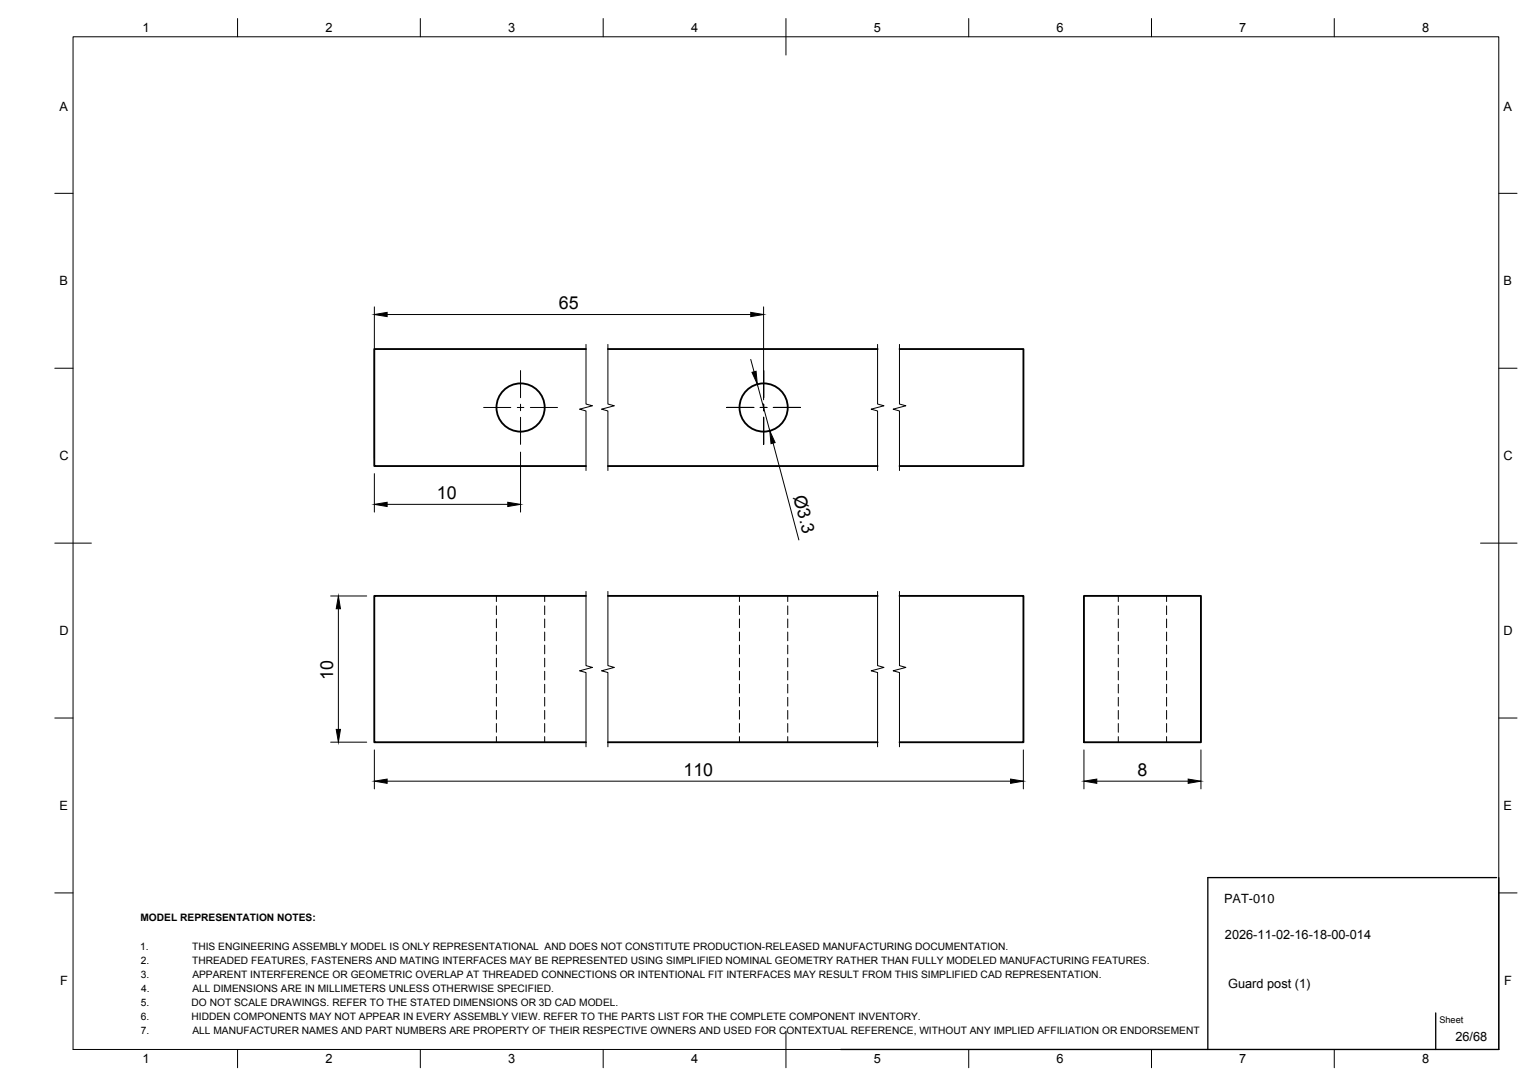
ISO-10303-21;
HEADER;
/* Generated by software containing ST-Developer
 * from STEP Tools, Inc. (www.steptools.com) 
 */

FILE_DESCRIPTION(
/* description */ ('Belt conveyor head drive unit'),
/* implementation_level */ '2;1');

FILE_NAME(
/* name */ 'Guard post (1).step',
/* time_stamp */ '2026-10-28T03:26:19-07:00',
/* author */ (''),
/* organization */ (''),
/* preprocessor_version */ 'ST-DEVELOPER v20.2',
/* originating_system */ 'Autodesk Translation Framework v15.17.0.0',
/* authorisation */ '');

FILE_SCHEMA (('AUTOMOTIVE_DESIGN { 1 0 10303 214 3 1 1 }'));
ENDSEC;

DATA;
#10=MECHANICAL_DESIGN_GEOMETRIC_PRESENTATION_REPRESENTATION('',(#872),#27069);
#734=SHAPE_REPRESENTATION_RELATIONSHIP('SRR','None',#27378,#803);
#803=ADVANCED_BREP_SHAPE_REPRESENTATION('',(#957),#27020);
#872=STYLED_ITEM('',(#27790),#957);
#957=MANIFOLD_SOLID_BREP('Body1',#13737);
#1139=FACE_BOUND('',#2847,.T.);
#1140=FACE_BOUND('',#2848,.T.);
#1141=FACE_BOUND('',#2851,.T.);
#1142=FACE_BOUND('',#2852,.T.);
#1425=PLANE('',#15164);
#1426=PLANE('',#15165);
#1427=PLANE('',#15166);
#1428=PLANE('',#15167);
#1429=PLANE('',#15168);
#1430=PLANE('',#15169);
#1917=FACE_OUTER_BOUND('',#2844,.T.);
#1918=FACE_OUTER_BOUND('',#2845,.T.);
#1919=FACE_OUTER_BOUND('',#2846,.T.);
#1920=FACE_OUTER_BOUND('',#2849,.T.);
#1921=FACE_OUTER_BOUND('',#2850,.T.);
#1922=FACE_OUTER_BOUND('',#2853,.T.);
#1923=FACE_OUTER_BOUND('',#2854,.T.);
#1924=FACE_OUTER_BOUND('',#2855,.T.);
#2844=EDGE_LOOP('',(#10188,#10189,#10190,#10191));
#2845=EDGE_LOOP('',(#10192,#10193,#10194,#10195));
#2846=EDGE_LOOP('',(#10196,#10197,#10198,#10199));
#2847=EDGE_LOOP('',(#10200));
#2848=EDGE_LOOP('',(#10201));
#2849=EDGE_LOOP('',(#10202,#10203,#10204,#10205));
#2850=EDGE_LOOP('',(#10206,#10207,#10208,#10209));
#2851=EDGE_LOOP('',(#10210));
#2852=EDGE_LOOP('',(#10211));
#2853=EDGE_LOOP('',(#10212,#10213,#10214,#10215));
#2854=EDGE_LOOP('',(#10216,#10217,#10218,#10219));
#2855=EDGE_LOOP('',(#10220,#10221,#10222,#10223));
#3829=LINE('',#22311,#4621);
#3830=LINE('',#22317,#4622);
#3831=LINE('',#22322,#4623);
#3832=LINE('',#22324,#4624);
#3833=LINE('',#22326,#4625);
#3834=LINE('',#22327,#4626);
#3835=LINE('',#22330,#4627);
#3836=LINE('',#22332,#4628);
#3837=LINE('',#22333,#4629);
#3838=LINE('',#22336,#4630);
#3839=LINE('',#22338,#4631);
#3840=LINE('',#22339,#4632);
#3841=LINE('',#22341,#4633);
#3842=LINE('',#22342,#4634);
#4621=VECTOR('',#17961,0.164999999999999);
#4622=VECTOR('',#17968,0.164999999999999);
#4623=VECTOR('',#17973,1.);
#4624=VECTOR('',#17974,1.);
#4625=VECTOR('',#17975,1.);
#4626=VECTOR('',#17976,1.);
#4627=VECTOR('',#17979,1.);
#4628=VECTOR('',#17980,1.);
#4629=VECTOR('',#17981,1.);
#4630=VECTOR('',#17984,1.);
#4631=VECTOR('',#17985,1.);
#4632=VECTOR('',#17986,1.);
#4633=VECTOR('',#17989,1.);
#4634=VECTOR('',#17990,1.);
#5366=CIRCLE('',#15159,0.164999999999999);
#5367=CIRCLE('',#15160,0.164999999999999);
#5368=CIRCLE('',#15162,0.164999999999999);
#5369=CIRCLE('',#15163,0.164999999999999);
#6363=VERTEX_POINT('',#22308);
#6364=VERTEX_POINT('',#22310);
#6365=VERTEX_POINT('',#22314);
#6366=VERTEX_POINT('',#22316);
#6367=VERTEX_POINT('',#22320);
#6368=VERTEX_POINT('',#22321);
#6369=VERTEX_POINT('',#22323);
#6370=VERTEX_POINT('',#22325);
#6371=VERTEX_POINT('',#22329);
#6372=VERTEX_POINT('',#22331);
#6373=VERTEX_POINT('',#22335);
#6374=VERTEX_POINT('',#22337);
#7786=EDGE_CURVE('',#6363,#6363,#5366,.T.);
#7787=EDGE_CURVE('',#6363,#6364,#3829,.T.);
#7788=EDGE_CURVE('',#6364,#6364,#5367,.T.);
#7789=EDGE_CURVE('',#6365,#6365,#5368,.T.);
#7790=EDGE_CURVE('',#6365,#6366,#3830,.T.);
#7791=EDGE_CURVE('',#6366,#6366,#5369,.T.);
#7792=EDGE_CURVE('',#6367,#6368,#3831,.T.);
#7793=EDGE_CURVE('',#6368,#6369,#3832,.T.);
#7794=EDGE_CURVE('',#6370,#6369,#3833,.T.);
#7795=EDGE_CURVE('',#6367,#6370,#3834,.T.);
#7796=EDGE_CURVE('',#6371,#6367,#3835,.T.);
#7797=EDGE_CURVE('',#6372,#6370,#3836,.T.);
#7798=EDGE_CURVE('',#6371,#6372,#3837,.T.);
#7799=EDGE_CURVE('',#6373,#6371,#3838,.T.);
#7800=EDGE_CURVE('',#6374,#6372,#3839,.T.);
#7801=EDGE_CURVE('',#6373,#6374,#3840,.T.);
#7802=EDGE_CURVE('',#6368,#6373,#3841,.T.);
#7803=EDGE_CURVE('',#6369,#6374,#3842,.T.);
#10188=ORIENTED_EDGE('',*,*,#7786,.F.);
#10189=ORIENTED_EDGE('',*,*,#7787,.T.);
#10190=ORIENTED_EDGE('',*,*,#7788,.F.);
#10191=ORIENTED_EDGE('',*,*,#7787,.F.);
#10192=ORIENTED_EDGE('',*,*,#7789,.F.);
#10193=ORIENTED_EDGE('',*,*,#7790,.T.);
#10194=ORIENTED_EDGE('',*,*,#7791,.F.);
#10195=ORIENTED_EDGE('',*,*,#7790,.F.);
#10196=ORIENTED_EDGE('',*,*,#7792,.T.);
#10197=ORIENTED_EDGE('',*,*,#7793,.T.);
#10198=ORIENTED_EDGE('',*,*,#7794,.F.);
#10199=ORIENTED_EDGE('',*,*,#7795,.F.);
#10200=ORIENTED_EDGE('',*,*,#7788,.T.);
#10201=ORIENTED_EDGE('',*,*,#7791,.T.);
#10202=ORIENTED_EDGE('',*,*,#7796,.T.);
#10203=ORIENTED_EDGE('',*,*,#7795,.T.);
#10204=ORIENTED_EDGE('',*,*,#7797,.F.);
#10205=ORIENTED_EDGE('',*,*,#7798,.F.);
#10206=ORIENTED_EDGE('',*,*,#7799,.T.);
#10207=ORIENTED_EDGE('',*,*,#7798,.T.);
#10208=ORIENTED_EDGE('',*,*,#7800,.F.);
#10209=ORIENTED_EDGE('',*,*,#7801,.F.);
#10210=ORIENTED_EDGE('',*,*,#7786,.T.);
#10211=ORIENTED_EDGE('',*,*,#7789,.T.);
#10212=ORIENTED_EDGE('',*,*,#7802,.T.);
#10213=ORIENTED_EDGE('',*,*,#7801,.T.);
#10214=ORIENTED_EDGE('',*,*,#7803,.F.);
#10215=ORIENTED_EDGE('',*,*,#7793,.F.);
#10216=ORIENTED_EDGE('',*,*,#7803,.T.);
#10217=ORIENTED_EDGE('',*,*,#7800,.T.);
#10218=ORIENTED_EDGE('',*,*,#7797,.T.);
#10219=ORIENTED_EDGE('',*,*,#7794,.T.);
#10220=ORIENTED_EDGE('',*,*,#7802,.F.);
#10221=ORIENTED_EDGE('',*,*,#7792,.F.);
#10222=ORIENTED_EDGE('',*,*,#7796,.F.);
#10223=ORIENTED_EDGE('',*,*,#7799,.F.);
#12668=CYLINDRICAL_SURFACE('',#15158,0.164999999999999);
#12669=CYLINDRICAL_SURFACE('',#15161,0.164999999999999);
#13196=ADVANCED_FACE('',(#1917),#12668,.F.);
#13197=ADVANCED_FACE('',(#1918),#12669,.F.);
#13198=ADVANCED_FACE('',(#1919,#1139,#1140),#1425,.T.);
#13199=ADVANCED_FACE('',(#1920),#1426,.T.);
#13200=ADVANCED_FACE('',(#1921,#1141,#1142),#1427,.T.);
#13201=ADVANCED_FACE('',(#1922),#1428,.T.);
#13202=ADVANCED_FACE('',(#1923),#1429,.T.);
#13203=ADVANCED_FACE('',(#1924),#1430,.F.);
#13737=CLOSED_SHELL('',(#13196,#13197,#13198,#13199,#13200,#13201,#13202,
#13203));
#15157=AXIS2_PLACEMENT_3D('',#22306,#17955,#17956);
#15158=AXIS2_PLACEMENT_3D('',#22307,#17957,#17958);
#15159=AXIS2_PLACEMENT_3D('',#22309,#17959,#17960);
#15160=AXIS2_PLACEMENT_3D('',#22312,#17962,#17963);
#15161=AXIS2_PLACEMENT_3D('',#22313,#17964,#17965);
#15162=AXIS2_PLACEMENT_3D('',#22315,#17966,#17967);
#15163=AXIS2_PLACEMENT_3D('',#22318,#17969,#17970);
#15164=AXIS2_PLACEMENT_3D('',#22319,#17971,#17972);
#15165=AXIS2_PLACEMENT_3D('',#22328,#17977,#17978);
#15166=AXIS2_PLACEMENT_3D('',#22334,#17982,#17983);
#15167=AXIS2_PLACEMENT_3D('',#22340,#17987,#17988);
#15168=AXIS2_PLACEMENT_3D('',#22343,#17991,#17992);
#15169=AXIS2_PLACEMENT_3D('',#22344,#17993,#17994);
#17955=DIRECTION('axis',(0.,0.,1.));
#17956=DIRECTION('refdir',(1.,0.,0.));
#17957=DIRECTION('center_axis',(0.,1.,0.));
#17958=DIRECTION('ref_axis',(1.,0.,0.));
#17959=DIRECTION('center_axis',(0.,1.,0.));
#17960=DIRECTION('ref_axis',(1.,0.,0.));
#17961=DIRECTION('',(0.,1.,0.));
#17962=DIRECTION('center_axis',(0.,-1.,0.));
#17963=DIRECTION('ref_axis',(1.,0.,0.));
#17964=DIRECTION('center_axis',(0.,1.,0.));
#17965=DIRECTION('ref_axis',(1.,0.,0.));
#17966=DIRECTION('center_axis',(0.,1.,0.));
#17967=DIRECTION('ref_axis',(1.,0.,0.));
#17968=DIRECTION('',(0.,1.,0.));
#17969=DIRECTION('center_axis',(0.,-1.,0.));
#17970=DIRECTION('ref_axis',(1.,0.,0.));
#17971=DIRECTION('center_axis',(0.,1.,0.));
#17972=DIRECTION('ref_axis',(-1.,0.,0.));
#17973=DIRECTION('',(-1.,0.,0.));
#17974=DIRECTION('',(0.,0.,1.));
#17975=DIRECTION('',(-1.,0.,0.));
#17976=DIRECTION('',(0.,0.,1.));
#17977=DIRECTION('center_axis',(1.,0.,0.));
#17978=DIRECTION('ref_axis',(0.,1.,0.));
#17979=DIRECTION('',(0.,1.,0.));
#17980=DIRECTION('',(0.,1.,0.));
#17981=DIRECTION('',(0.,0.,1.));
#17982=DIRECTION('center_axis',(0.,-1.,0.));
#17983=DIRECTION('ref_axis',(1.,0.,0.));
#17984=DIRECTION('',(1.,0.,0.));
#17985=DIRECTION('',(1.,0.,0.));
#17986=DIRECTION('',(0.,0.,1.));
#17987=DIRECTION('center_axis',(-1.,0.,0.));
#17988=DIRECTION('ref_axis',(0.,-1.,0.));
#17989=DIRECTION('',(0.,-1.,0.));
#17990=DIRECTION('',(0.,-1.,0.));
#17991=DIRECTION('center_axis',(0.,0.,1.));
#17992=DIRECTION('ref_axis',(1.,0.,0.));
#17993=DIRECTION('center_axis',(0.,0.,1.));
#17994=DIRECTION('ref_axis',(1.,0.,0.));
#22306=CARTESIAN_POINT('',(0.,0.,0.));
#22307=CARTESIAN_POINT('Origin',(9.97091003018116,-6.1,4.5));
#22308=CARTESIAN_POINT('',(9.80591003018116,-6.,4.5));
#22309=CARTESIAN_POINT('Origin',(9.97091003018116,-6.,4.5));
#22310=CARTESIAN_POINT('',(9.80591003018116,-5.,4.5));
#22311=CARTESIAN_POINT('',(9.80591003018116,-6.1,4.5));
#22312=CARTESIAN_POINT('Origin',(9.97091003018116,-5.,4.5));
#22313=CARTESIAN_POINT('Origin',(9.97091003018116,-6.1,10.));
#22314=CARTESIAN_POINT('',(9.80591003018116,-6.,10.));
#22315=CARTESIAN_POINT('Origin',(9.97091003018116,-6.,10.));
#22316=CARTESIAN_POINT('',(9.80591003018116,-5.,10.));
#22317=CARTESIAN_POINT('',(9.80591003018116,-6.1,10.));
#22318=CARTESIAN_POINT('Origin',(9.97091003018116,-5.,10.));
#22319=CARTESIAN_POINT('Origin',(10.3709100301812,-5.,0.));
#22320=CARTESIAN_POINT('',(10.3709100301812,-5.,0.));
#22321=CARTESIAN_POINT('',(9.57091003018116,-5.,0.));
#22322=CARTESIAN_POINT('',(10.3709100301812,-5.,0.));
#22323=CARTESIAN_POINT('',(9.57091003018116,-5.,11.));
#22324=CARTESIAN_POINT('',(9.57091003018116,-5.,0.));
#22325=CARTESIAN_POINT('',(10.3709100301812,-5.,11.));
#22326=CARTESIAN_POINT('',(10.3709100301812,-5.,11.));
#22327=CARTESIAN_POINT('',(10.3709100301812,-5.,0.));
#22328=CARTESIAN_POINT('Origin',(10.3709100301812,-6.,0.));
#22329=CARTESIAN_POINT('',(10.3709100301812,-6.,0.));
#22330=CARTESIAN_POINT('',(10.3709100301812,-6.,0.));
#22331=CARTESIAN_POINT('',(10.3709100301812,-6.,11.));
#22332=CARTESIAN_POINT('',(10.3709100301812,-6.,11.));
#22333=CARTESIAN_POINT('',(10.3709100301812,-6.,0.));
#22334=CARTESIAN_POINT('Origin',(9.57091003018116,-6.,0.));
#22335=CARTESIAN_POINT('',(9.57091003018116,-6.,0.));
#22336=CARTESIAN_POINT('',(9.57091003018116,-6.,0.));
#22337=CARTESIAN_POINT('',(9.57091003018116,-6.,11.));
#22338=CARTESIAN_POINT('',(9.57091003018116,-6.,11.));
#22339=CARTESIAN_POINT('',(9.57091003018116,-6.,0.));
#22340=CARTESIAN_POINT('Origin',(9.57091003018116,-5.,0.));
#22341=CARTESIAN_POINT('',(9.57091003018116,-5.,0.));
#22342=CARTESIAN_POINT('',(9.57091003018116,-5.,11.));
#22343=CARTESIAN_POINT('Origin',(9.97091003018116,-5.5,11.));
#22344=CARTESIAN_POINT('Origin',(9.97091003018116,-5.5,0.));
#26943=UNCERTAINTY_MEASURE_WITH_UNIT(LENGTH_MEASURE(0.001),#27070,
'DISTANCE_ACCURACY_VALUE',
'Maximum model space distance between geometric entities at asserted c
onnectivities');
#26992=UNCERTAINTY_MEASURE_WITH_UNIT(LENGTH_MEASURE(0.001),#27070,
'DISTANCE_ACCURACY_VALUE',
'Maximum model space distance between geometric entities at asserted c
onnectivities');
#27020=(
GEOMETRIC_REPRESENTATION_CONTEXT(3)
GLOBAL_UNCERTAINTY_ASSIGNED_CONTEXT((#26943))
GLOBAL_UNIT_ASSIGNED_CONTEXT((#27070,#27072,#27073))
REPRESENTATION_CONTEXT('','3D')
);
#27069=(
GEOMETRIC_REPRESENTATION_CONTEXT(3)
GLOBAL_UNCERTAINTY_ASSIGNED_CONTEXT((#26992))
GLOBAL_UNIT_ASSIGNED_CONTEXT((#27070,#27072,#27073))
REPRESENTATION_CONTEXT('','3D')
);
#27070=(
LENGTH_UNIT()
NAMED_UNIT(*)
SI_UNIT(.CENTI.,.METRE.)
);
#27072=(
NAMED_UNIT(*)
PLANE_ANGLE_UNIT()
SI_UNIT($,.RADIAN.)
);
#27073=(
NAMED_UNIT(*)
SI_UNIT($,.STERADIAN.)
SOLID_ANGLE_UNIT()
);
#27101=SHAPE_DEFINITION_REPRESENTATION(#27177,#27378);
#27177=PRODUCT_DEFINITION_SHAPE('',$,#27455);
#27378=SHAPE_REPRESENTATION('',(#15157),#27020);
#27427=PRODUCT_DEFINITION_CONTEXT('part definition',#27657,'design');
#27455=PRODUCT_DEFINITION('Guard post (1)','Guard post (1)',#27531,#27427);
#27531=PRODUCT_DEFINITION_FORMATION('',$,#27686);
#27657=APPLICATION_CONTEXT(
'Core Data for Automotive Mechanical Design Process');
#27658=PRODUCT_CONTEXT('part definition',#27657,'mechanical');
#27686=PRODUCT('Guard post (1)','Guard post (1)','Guard post (1)',(#27658));
#27784=COLOUR_RGB('Sky Blue',0.24,0.69,0.87);
#27785=FILL_AREA_STYLE_COLOUR('',#27784);
#27786=FILL_AREA_STYLE('',(#27785));
#27787=SURFACE_STYLE_FILL_AREA(#27786);
#27788=SURFACE_SIDE_STYLE('',(#27787));
#27789=SURFACE_STYLE_USAGE(.BOTH.,#27788);
#27790=PRESENTATION_STYLE_ASSIGNMENT((#27789));
ENDSEC;
END-ISO-10303-21;
